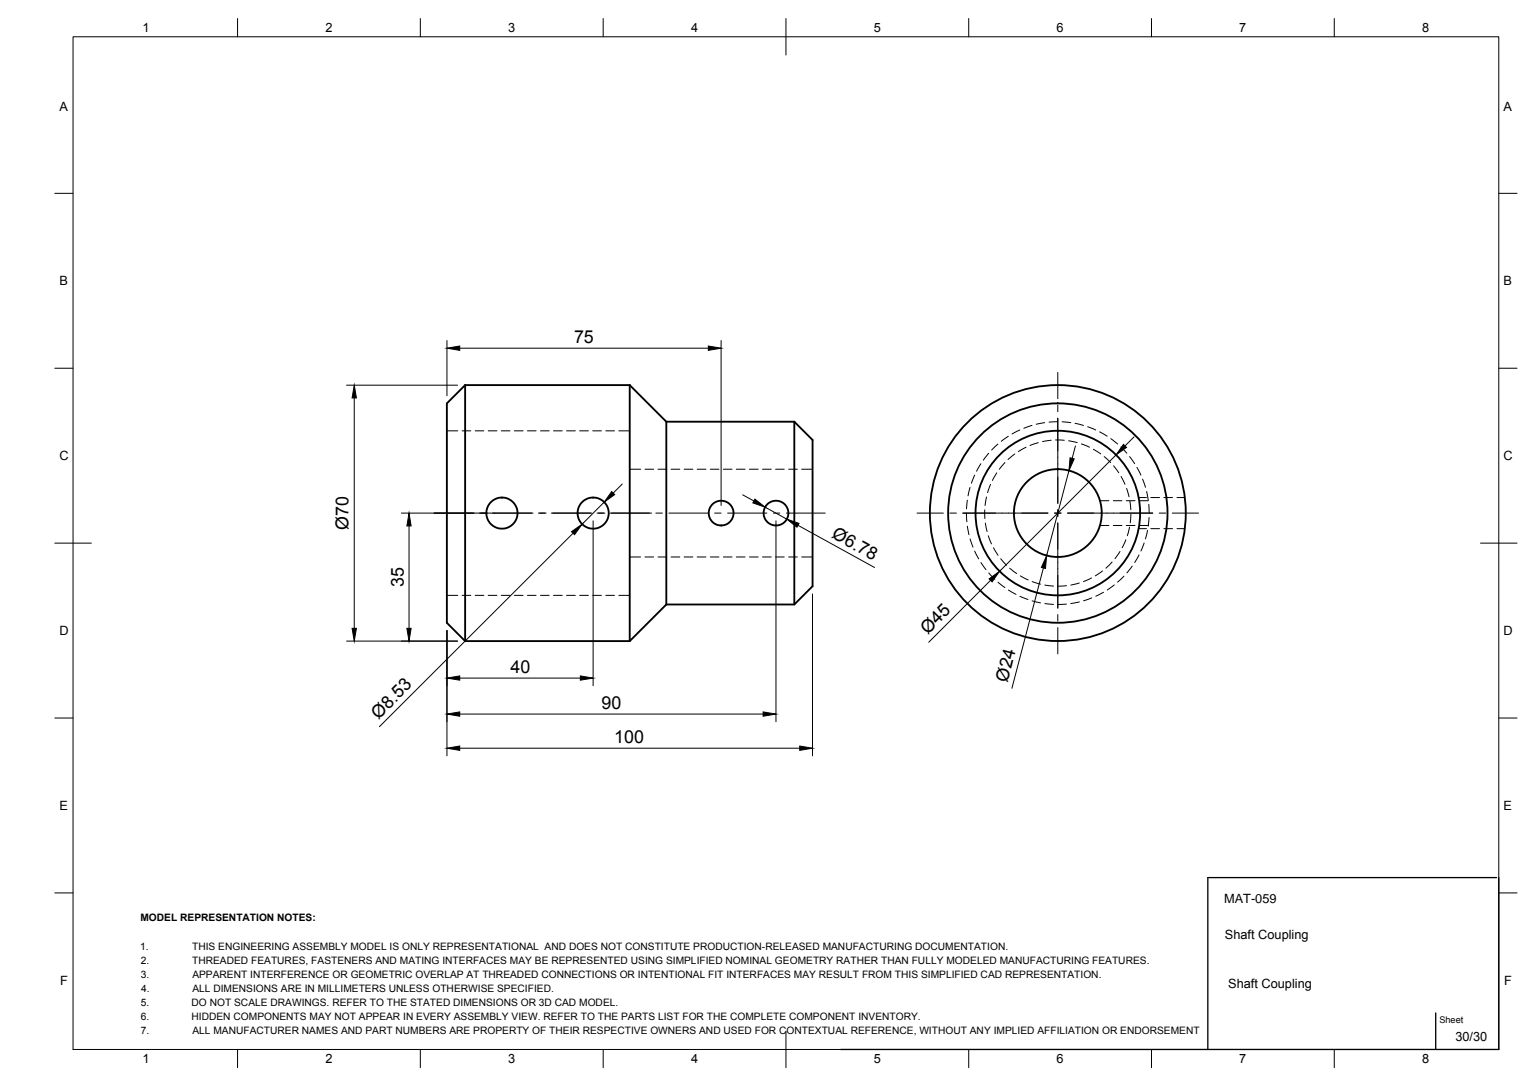
ISO-10303-21;
HEADER;
/* Generated by software containing ST-Developer
 * from STEP Tools, Inc. (www.steptools.com) 
 */

FILE_DESCRIPTION(
/* description */ ('', 'CAx-IF Rec.Pracs.---Representation and Presentation of Product Manufa
cturing Information (PMI)---4.0---2014-10-13'),
/* implementation_level */ '2;1');

FILE_NAME(
/* name */ 'Shaft Coupling.step',
/* time_stamp */ '2026-10-28T23:00:48+01:00',
/* author */ (''),
/* organization */ (''),
/* preprocessor_version */ 'ST-DEVELOPER v20.2',
/* originating_system */ 'Autodesk Translation Framework v15.17.0.0',
/* authorisation */ '');

FILE_SCHEMA (('AP242_MANAGED_MODEL_BASED_3D_ENGINEERING_MIM_LF { 1 0 10303 442 2 1 4 }'));
ENDSEC;

DATA;
#10=MECHANICAL_DESIGN_GEOMETRIC_PRESENTATION_REPRESENTATION('',(#999),#61811);
#707=CONICAL_SURFACE('',#38104,20.4999999999999,0.785398163397433);
#708=CONICAL_SURFACE('',#38107,30.4999999999998,0.785398163397455);
#709=CONICAL_SURFACE('',#38115,26.0000000000003,0.785398163397453);
#844=B_SPLINE_CURVE_WITH_KNOTS('',3,(#61360,#61361,#61362,#61363,#61364,
#61365,#61366,#61367,#61368,#61369,#61370,#61371,#61372,#61373,#61374,#61375,
#61376,#61377,#61378,#61379,#61380,#61381,#61382,#61383,#61384,#61385,#61386,
#61387,#61388,#61389,#61390,#61391,#61392,#61393),.UNSPECIFIED.,.T.,.F.,
(4,2,2,2,2,2,2,2,2,2,2,2,2,2,2,2,4),(-2.05511901424686,-1.92665918665082,
-1.79819935905478,-1.66976930986996,-1.54133926068514,-1.41290921150033,
-1.28447916231551,-1.15601933471947,-1.02755950712343,-0.899099679527391,
-0.770639851931354,-0.642209802746534,-0.513779753561715,-0.385349704376896,
-0.256919655192076,-0.128459827596038,0.),.UNSPECIFIED.);
#845=B_SPLINE_CURVE_WITH_KNOTS('',3,(#61395,#61396,#61397,#61398,#61399,
#61400,#61401,#61402,#61403,#61404,#61405,#61406,#61407,#61408,#61409,#61410,
#61411,#61412,#61413,#61414,#61415,#61416,#61417,#61418,#61419,#61420,#61421,
#61422,#61423,#61424,#61425,#61426,#61427,#61428),.UNSPECIFIED.,.T.,.F.,
(4,2,2,2,2,2,2,2,2,2,2,2,2,2,2,2,4),(-2.05511901424684,-1.9266591866508,
-1.79819935905477,-1.66976930986995,-1.54133926068513,-1.41290921150031,
-1.2844791623155,-1.15601933471946,-1.02755950712342,-0.899099679527382,
-0.770639851931344,-0.642209802746527,-0.513779753561709,-0.385349704376891,
-0.256919655192072,-0.128459827596036,0.),.UNSPECIFIED.);
#846=B_SPLINE_CURVE_WITH_KNOTS('',3,(#61431,#61432,#61433,#61434,#61435,
#61436,#61437,#61438,#61439,#61440,#61441,#61442,#61443,#61444,#61445,#61446,
#61447,#61448,#61449,#61450,#61451,#61452,#61453,#61454,#61455,#61456,#61457,
#61458,#61459,#61460,#61461,#61462,#61463,#61464),.UNSPECIFIED.,.T.,.F.,
(4,2,2,2,2,2,2,2,2,2,2,2,2,2,2,2,4),(-2.57601194234862,-2.41500757713331,
-2.254003211918,-2.09300608433973,-1.93200895676147,-1.7710118291832,-1.61001470160494,
-1.44901033638962,-1.28800597117431,-1.127001605959,-0.965997240743687,
-0.805000113165422,-0.644002985587156,-0.483005858008892,-0.322008730430627,
-0.161004365215313,0.),.UNSPECIFIED.);
#847=B_SPLINE_CURVE_WITH_KNOTS('',3,(#61467,#61468,#61469,#61470,#61471,
#61472,#61473,#61474,#61475,#61476,#61477,#61478,#61479,#61480,#61481,#61482,
#61483,#61484,#61485,#61486,#61487,#61488,#61489,#61490,#61491,#61492,#61493,
#61494,#61495,#61496,#61497,#61498,#61499,#61500),.UNSPECIFIED.,.T.,.F.,
(4,2,2,2,2,2,2,2,2,2,2,2,2,2,2,2,4),(0.,0.160753606357945,0.321507212715889,
0.4822596093528,0.643012005989711,0.803764402626621,0.964516799263531,1.12527040562148,
1.28602401197942,1.44677761833737,1.60753122469531,1.76828362133222,1.92903601796913,
2.08978841460604,2.25054081124296,2.4112944176009,2.57204802395885),
 .UNSPECIFIED.);
#848=B_SPLINE_CURVE_WITH_KNOTS('',3,(#61503,#61504,#61505,#61506,#61507,
#61508,#61509,#61510,#61511,#61512,#61513,#61514,#61515,#61516,#61517,#61518,
#61519,#61520,#61521,#61522,#61523,#61524,#61525,#61526,#61527,#61528,#61529,
#61530,#61531,#61532,#61533,#61534,#61535,#61536),.UNSPECIFIED.,.T.,.F.,
(4,2,2,2,2,2,2,2,2,2,2,2,2,2,2,2,4),(-2.57601194234859,-2.41500757713328,
-2.25400321191797,-2.09300608433971,-1.93200895676145,-1.77101182918318,
-1.61001470160492,-1.44901033638961,-1.2880059711743,-1.12700160595899,
-0.965997240743677,-0.805000113165413,-0.644002985587149,-0.483005858008886,
-0.322008730430623,-0.161004365215312,0.),.UNSPECIFIED.);
#849=B_SPLINE_CURVE_WITH_KNOTS('',3,(#61539,#61540,#61541,#61542,#61543,
#61544,#61545,#61546,#61547,#61548,#61549,#61550,#61551,#61552,#61553,#61554,
#61555,#61556,#61557,#61558,#61559,#61560,#61561,#61562,#61563,#61564,#61565,
#61566,#61567,#61568,#61569,#61570,#61571,#61572),.UNSPECIFIED.,.T.,.F.,
(4,2,2,2,2,2,2,2,2,2,2,2,2,2,2,2,4),(0.,0.160753606357943,0.321507212715886,
0.482259609352795,0.643012005989704,0.803764402626612,0.964516799263521,
1.12527040562146,1.28602401197941,1.44677761833735,1.60753122469529,1.7682836213322,
1.92903601796911,2.08978841460602,2.25054081124293,2.41129441760087,2.57204802395882),
 .UNSPECIFIED.);
#850=B_SPLINE_CURVE_WITH_KNOTS('',3,(#61577,#61578,#61579,#61580,#61581,
#61582,#61583,#61584,#61585,#61586,#61587,#61588,#61589,#61590,#61591,#61592,
#61593,#61594),.UNSPECIFIED.,.F.,.F.,(4,2,2,2,2,2,2,2,4),(0.,0.127857366097431,
0.255714732194861,0.383570615681227,0.511426499167593,0.639282382653959,
0.767138266140325,0.894995632237756,1.02285299833519),.UNSPECIFIED.);
#851=B_SPLINE_CURVE_WITH_KNOTS('',3,(#61595,#61596,#61597,#61598,#61599,
#61600,#61601,#61602,#61603,#61604,#61605,#61606,#61607,#61608,#61609,#61610,
#61611,#61612),.UNSPECIFIED.,.F.,.F.,(4,2,2,2,2,2,2,2,4),(1.02285299833519,
1.15071036443262,1.27856773053005,1.40642361401641,1.53427949750278,1.66213538098915,
1.78999126447551,1.91784863057294,2.04570599667037),.UNSPECIFIED.);
#852=B_SPLINE_CURVE_WITH_KNOTS('',3,(#61617,#61618,#61619,#61620,#61621,
#61622,#61623,#61624,#61625,#61626,#61627,#61628,#61629,#61630,#61631,#61632,
#61633,#61634),.UNSPECIFIED.,.F.,.F.,(4,2,2,2,2,2,2,2,4),(0.,0.12785736609743,
0.255714732194861,0.383570615681225,0.511426499167589,0.639282382653953,
0.767138266140317,0.894995632237748,1.02285299833518),.UNSPECIFIED.);
#853=B_SPLINE_CURVE_WITH_KNOTS('',3,(#61635,#61636,#61637,#61638,#61639,
#61640,#61641,#61642,#61643,#61644,#61645,#61646,#61647,#61648,#61649,#61650,
#61651,#61652),.UNSPECIFIED.,.F.,.F.,(4,2,2,2,2,2,2,2,4),(1.02285299833518,
1.15071036443261,1.27856773053004,1.4064236140164,1.53427949750277,1.66213538098913,
1.7899912644755,1.91784863057293,2.04570599667036),.UNSPECIFIED.);
#935=SHAPE_REPRESENTATION_RELATIONSHIP('SRR','None',#61997,#960);
#960=ADVANCED_BREP_SHAPE_REPRESENTATION('',(#1037),#61810);
#999=STYLED_ITEM('',(#62156),#1037);
#1037=MANIFOLD_SOLID_BREP('Body1',#33839);
#1870=CYLINDRICAL_SURFACE('',#38088,12.);
#1871=CYLINDRICAL_SURFACE('',#38091,4.26299999999998);
#1872=CYLINDRICAL_SURFACE('',#38092,4.26299999999993);
#1873=CYLINDRICAL_SURFACE('',#38093,3.38975000000002);
#1874=CYLINDRICAL_SURFACE('',#38094,3.38974999999999);
#1875=CYLINDRICAL_SURFACE('',#38097,22.5);
#1876=CYLINDRICAL_SURFACE('',#38099,24.9999999999999);
#1877=CYLINDRICAL_SURFACE('',#38111,35.0000000000001);
#2225=FACE_BOUND('',#8322,.T.);
#2226=FACE_BOUND('',#8323,.T.);
#2227=FACE_BOUND('',#8329,.T.);
#2228=FACE_BOUND('',#8331,.T.);
#2229=FACE_BOUND('',#8332,.T.);
#2230=FACE_BOUND('',#8334,.T.);
#2231=FACE_BOUND('',#8335,.T.);
#2232=FACE_BOUND('',#8338,.T.);
#2233=FACE_BOUND('',#8341,.T.);
#2234=FACE_BOUND('',#8342,.T.);
#2235=FACE_BOUND('',#8344,.T.);
#4218=CIRCLE('',#38089,12.);
#4219=CIRCLE('',#38090,12.);
#4220=CIRCLE('',#38096,22.5);
#4221=CIRCLE('',#38098,22.5);
#4222=CIRCLE('',#38100,25.);
#4223=CIRCLE('',#38101,25.);
#4224=CIRCLE('',#38102,25.);
#4225=CIRCLE('',#38103,25.);
#4226=CIRCLE('',#38105,20.);
#4227=CIRCLE('',#38108,35.);
#4228=CIRCLE('',#38109,35.);
#4229=CIRCLE('',#38110,29.9999999999998);
#4230=CIRCLE('',#38112,35.0000000000001);
#4231=CIRCLE('',#38113,35.0000000000001);
#6096=FACE_OUTER_BOUND('',#8321,.T.);
#6097=FACE_OUTER_BOUND('',#8324,.T.);
#6098=FACE_OUTER_BOUND('',#8325,.T.);
#6099=FACE_OUTER_BOUND('',#8326,.T.);
#6100=FACE_OUTER_BOUND('',#8327,.T.);
#6101=FACE_OUTER_BOUND('',#8328,.T.);
#6102=FACE_OUTER_BOUND('',#8330,.T.);
#6103=FACE_OUTER_BOUND('',#8333,.T.);
#6104=FACE_OUTER_BOUND('',#8336,.T.);
#6105=FACE_OUTER_BOUND('',#8337,.T.);
#6106=FACE_OUTER_BOUND('',#8339,.T.);
#6107=FACE_OUTER_BOUND('',#8340,.T.);
#6108=FACE_OUTER_BOUND('',#8343,.T.);
#6109=FACE_OUTER_BOUND('',#8345,.T.);
#8321=EDGE_LOOP('',(#31042,#31043,#31044,#31045));
#8322=EDGE_LOOP('',(#31046));
#8323=EDGE_LOOP('',(#31047));
#8324=EDGE_LOOP('',(#31048,#31049,#31050,#31051));
#8325=EDGE_LOOP('',(#31052,#31053,#31054,#31055));
#8326=EDGE_LOOP('',(#31056,#31057,#31058,#31059,#31060));
#8327=EDGE_LOOP('',(#31061,#31062,#31063,#31064,#31065));
#8328=EDGE_LOOP('',(#31066));
#8329=EDGE_LOOP('',(#31067));
#8330=EDGE_LOOP('',(#31068,#31069,#31070,#31071));
#8331=EDGE_LOOP('',(#31072));
#8332=EDGE_LOOP('',(#31073));
#8333=EDGE_LOOP('',(#31074,#31075,#31076,#31077,#31078,#31079));
#8334=EDGE_LOOP('',(#31080,#31081));
#8335=EDGE_LOOP('',(#31082,#31083));
#8336=EDGE_LOOP('',(#31084,#31085,#31086,#31087,#31088));
#8337=EDGE_LOOP('',(#31089));
#8338=EDGE_LOOP('',(#31090));
#8339=EDGE_LOOP('',(#31091,#31092,#31093,#31094,#31095));
#8340=EDGE_LOOP('',(#31096,#31097,#31098,#31099,#31100,#31101));
#8341=EDGE_LOOP('',(#31102));
#8342=EDGE_LOOP('',(#31103));
#8343=EDGE_LOOP('',(#31104));
#8344=EDGE_LOOP('',(#31105));
#8345=EDGE_LOOP('',(#31106,#31107,#31108,#31109,#31110,#31111));
#10882=LINE('',#61357,#13429);
#10883=LINE('',#61466,#13430);
#10884=LINE('',#61538,#13431);
#10885=LINE('',#61575,#13432);
#10886=LINE('',#61615,#13433);
#10887=LINE('',#61658,#13434);
#10888=LINE('',#61666,#13435);
#10889=LINE('',#61672,#13436);
#10890=LINE('',#61681,#13437);
#10891=LINE('',#61685,#13438);
#10892=LINE('',#61691,#13439);
#13429=VECTOR('',#48658,12.);
#13430=VECTOR('',#48663,4.26299999999998);
#13431=VECTOR('',#48666,4.26299999999993);
#13432=VECTOR('',#48669,3.38975000000002);
#13433=VECTOR('',#48672,3.38974999999999);
#13434=VECTOR('',#48679,22.5);
#13435=VECTOR('',#48688,24.9999999999999);
#13436=VECTOR('',#48695,20.4999999999999);
#13437=VECTOR('',#48706,30.4999999999998);
#13438=VECTOR('',#48711,35.0000000000001);
#13439=VECTOR('',#48720,26.0000000000003);
#16607=VERTEX_POINT('',#61354);
#16608=VERTEX_POINT('',#61356);
#16609=VERTEX_POINT('',#61359);
#16610=VERTEX_POINT('',#61394);
#16611=VERTEX_POINT('',#61430);
#16612=VERTEX_POINT('',#61465);
#16613=VERTEX_POINT('',#61502);
#16614=VERTEX_POINT('',#61537);
#16615=VERTEX_POINT('',#61574);
#16616=VERTEX_POINT('',#61576);
#16617=VERTEX_POINT('',#61614);
#16618=VERTEX_POINT('',#61616);
#16619=VERTEX_POINT('',#61654);
#16620=VERTEX_POINT('',#61657);
#16621=VERTEX_POINT('',#61661);
#16622=VERTEX_POINT('',#61662);
#16623=VERTEX_POINT('',#61665);
#16624=VERTEX_POINT('',#61667);
#16625=VERTEX_POINT('',#61671);
#16626=VERTEX_POINT('',#61676);
#16627=VERTEX_POINT('',#61677);
#16628=VERTEX_POINT('',#61680);
#16629=VERTEX_POINT('',#61684);
#16630=VERTEX_POINT('',#61686);
#21423=EDGE_CURVE('',#16607,#16607,#4218,.T.);
#21424=EDGE_CURVE('',#16607,#16608,#10882,.T.);
#21425=EDGE_CURVE('',#16608,#16608,#4219,.T.);
#21426=EDGE_CURVE('',#16609,#16609,#844,.T.);
#21427=EDGE_CURVE('',#16610,#16610,#845,.T.);
#21428=EDGE_CURVE('',#16611,#16611,#846,.T.);
#21429=EDGE_CURVE('',#16611,#16612,#10883,.T.);
#21430=EDGE_CURVE('',#16612,#16612,#847,.T.);
#21431=EDGE_CURVE('',#16613,#16613,#848,.T.);
#21432=EDGE_CURVE('',#16613,#16614,#10884,.T.);
#21433=EDGE_CURVE('',#16614,#16614,#849,.T.);
#21434=EDGE_CURVE('',#16609,#16615,#10885,.T.);
#21435=EDGE_CURVE('',#16616,#16615,#850,.T.);
#21436=EDGE_CURVE('',#16615,#16616,#851,.T.);
#21437=EDGE_CURVE('',#16610,#16617,#10886,.T.);
#21438=EDGE_CURVE('',#16618,#16617,#852,.T.);
#21439=EDGE_CURVE('',#16617,#16618,#853,.T.);
#21440=EDGE_CURVE('',#16619,#16619,#4220,.T.);
#21441=EDGE_CURVE('',#16619,#16620,#10887,.T.);
#21442=EDGE_CURVE('',#16620,#16620,#4221,.T.);
#21443=EDGE_CURVE('',#16621,#16622,#4222,.T.);
#21444=EDGE_CURVE('',#16622,#16621,#4223,.T.);
#21445=EDGE_CURVE('',#16622,#16623,#10888,.T.);
#21446=EDGE_CURVE('',#16624,#16623,#4224,.T.);
#21447=EDGE_CURVE('',#16623,#16624,#4225,.T.);
#21448=EDGE_CURVE('',#16621,#16625,#10889,.T.);
#21449=EDGE_CURVE('',#16625,#16625,#4226,.T.);
#21450=EDGE_CURVE('',#16626,#16627,#4227,.T.);
#21451=EDGE_CURVE('',#16627,#16626,#4228,.T.);
#21452=EDGE_CURVE('',#16626,#16628,#10890,.T.);
#21453=EDGE_CURVE('',#16628,#16628,#4229,.T.);
#21454=EDGE_CURVE('',#16627,#16629,#10891,.T.);
#21455=EDGE_CURVE('',#16630,#16629,#4230,.T.);
#21456=EDGE_CURVE('',#16629,#16630,#4231,.T.);
#21457=EDGE_CURVE('',#16630,#16624,#10892,.T.);
#31042=ORIENTED_EDGE('',*,*,#21423,.F.);
#31043=ORIENTED_EDGE('',*,*,#21424,.T.);
#31044=ORIENTED_EDGE('',*,*,#21425,.F.);
#31045=ORIENTED_EDGE('',*,*,#21424,.F.);
#31046=ORIENTED_EDGE('',*,*,#21426,.F.);
#31047=ORIENTED_EDGE('',*,*,#21427,.F.);
#31048=ORIENTED_EDGE('',*,*,#21428,.F.);
#31049=ORIENTED_EDGE('',*,*,#21429,.T.);
#31050=ORIENTED_EDGE('',*,*,#21430,.F.);
#31051=ORIENTED_EDGE('',*,*,#21429,.F.);
#31052=ORIENTED_EDGE('',*,*,#21431,.F.);
#31053=ORIENTED_EDGE('',*,*,#21432,.T.);
#31054=ORIENTED_EDGE('',*,*,#21433,.F.);
#31055=ORIENTED_EDGE('',*,*,#21432,.F.);
#31056=ORIENTED_EDGE('',*,*,#21426,.T.);
#31057=ORIENTED_EDGE('',*,*,#21434,.T.);
#31058=ORIENTED_EDGE('',*,*,#21435,.F.);
#31059=ORIENTED_EDGE('',*,*,#21436,.F.);
#31060=ORIENTED_EDGE('',*,*,#21434,.F.);
#31061=ORIENTED_EDGE('',*,*,#21427,.T.);
#31062=ORIENTED_EDGE('',*,*,#21437,.T.);
#31063=ORIENTED_EDGE('',*,*,#21438,.F.);
#31064=ORIENTED_EDGE('',*,*,#21439,.F.);
#31065=ORIENTED_EDGE('',*,*,#21437,.F.);
#31066=ORIENTED_EDGE('',*,*,#21440,.T.);
#31067=ORIENTED_EDGE('',*,*,#21425,.T.);
#31068=ORIENTED_EDGE('',*,*,#21440,.F.);
#31069=ORIENTED_EDGE('',*,*,#21441,.T.);
#31070=ORIENTED_EDGE('',*,*,#21442,.F.);
#31071=ORIENTED_EDGE('',*,*,#21441,.F.);
#31072=ORIENTED_EDGE('',*,*,#21428,.T.);
#31073=ORIENTED_EDGE('',*,*,#21431,.T.);
#31074=ORIENTED_EDGE('',*,*,#21443,.F.);
#31075=ORIENTED_EDGE('',*,*,#21444,.F.);
#31076=ORIENTED_EDGE('',*,*,#21445,.T.);
#31077=ORIENTED_EDGE('',*,*,#21446,.F.);
#31078=ORIENTED_EDGE('',*,*,#21447,.F.);
#31079=ORIENTED_EDGE('',*,*,#21445,.F.);
#31080=ORIENTED_EDGE('',*,*,#21435,.T.);
#31081=ORIENTED_EDGE('',*,*,#21436,.T.);
#31082=ORIENTED_EDGE('',*,*,#21438,.T.);
#31083=ORIENTED_EDGE('',*,*,#21439,.T.);
#31084=ORIENTED_EDGE('',*,*,#21443,.T.);
#31085=ORIENTED_EDGE('',*,*,#21444,.T.);
#31086=ORIENTED_EDGE('',*,*,#21448,.T.);
#31087=ORIENTED_EDGE('',*,*,#21449,.T.);
#31088=ORIENTED_EDGE('',*,*,#21448,.F.);
#31089=ORIENTED_EDGE('',*,*,#21449,.F.);
#31090=ORIENTED_EDGE('',*,*,#21423,.T.);
#31091=ORIENTED_EDGE('',*,*,#21450,.T.);
#31092=ORIENTED_EDGE('',*,*,#21451,.T.);
#31093=ORIENTED_EDGE('',*,*,#21452,.T.);
#31094=ORIENTED_EDGE('',*,*,#21453,.T.);
#31095=ORIENTED_EDGE('',*,*,#21452,.F.);
#31096=ORIENTED_EDGE('',*,*,#21450,.F.);
#31097=ORIENTED_EDGE('',*,*,#21451,.F.);
#31098=ORIENTED_EDGE('',*,*,#21454,.T.);
#31099=ORIENTED_EDGE('',*,*,#21455,.F.);
#31100=ORIENTED_EDGE('',*,*,#21456,.F.);
#31101=ORIENTED_EDGE('',*,*,#21454,.F.);
#31102=ORIENTED_EDGE('',*,*,#21430,.T.);
#31103=ORIENTED_EDGE('',*,*,#21433,.T.);
#31104=ORIENTED_EDGE('',*,*,#21453,.F.);
#31105=ORIENTED_EDGE('',*,*,#21442,.T.);
#31106=ORIENTED_EDGE('',*,*,#21456,.T.);
#31107=ORIENTED_EDGE('',*,*,#21457,.T.);
#31108=ORIENTED_EDGE('',*,*,#21446,.T.);
#31109=ORIENTED_EDGE('',*,*,#21447,.T.);
#31110=ORIENTED_EDGE('',*,*,#21457,.F.);
#31111=ORIENTED_EDGE('',*,*,#21455,.T.);
#31910=PLANE('',#38095);
#31911=PLANE('',#38106);
#31912=PLANE('',#38114);
#33777=ADVANCED_FACE('',(#6096,#2225,#2226),#1870,.F.);
#33778=ADVANCED_FACE('',(#6097),#1871,.F.);
#33779=ADVANCED_FACE('',(#6098),#1872,.F.);
#33780=ADVANCED_FACE('',(#6099),#1873,.F.);
#33781=ADVANCED_FACE('',(#6100),#1874,.F.);
#33782=ADVANCED_FACE('',(#6101,#2227),#31910,.T.);
#33783=ADVANCED_FACE('',(#6102,#2228,#2229),#1875,.F.);
#33784=ADVANCED_FACE('',(#6103,#2230,#2231),#1876,.T.);
#33785=ADVANCED_FACE('',(#6104),#707,.T.);
#33786=ADVANCED_FACE('',(#6105,#2232),#31911,.T.);
#33787=ADVANCED_FACE('',(#6106),#708,.T.);
#33788=ADVANCED_FACE('',(#6107,#2233,#2234),#1877,.T.);
#33789=ADVANCED_FACE('',(#6108,#2235),#31912,.T.);
#33790=ADVANCED_FACE('',(#6109),#709,.T.);
#33839=CLOSED_SHELL('',(#33777,#33778,#33779,#33780,#33781,#33782,#33783,
#33784,#33785,#33786,#33787,#33788,#33789,#33790));
#38087=AXIS2_PLACEMENT_3D('',#61352,#48652,#48653);
#38088=AXIS2_PLACEMENT_3D('',#61353,#48654,#48655);
#38089=AXIS2_PLACEMENT_3D('',#61355,#48656,#48657);
#38090=AXIS2_PLACEMENT_3D('',#61358,#48659,#48660);
#38091=AXIS2_PLACEMENT_3D('',#61429,#48661,#48662);
#38092=AXIS2_PLACEMENT_3D('',#61501,#48664,#48665);
#38093=AXIS2_PLACEMENT_3D('',#61573,#48667,#48668);
#38094=AXIS2_PLACEMENT_3D('',#61613,#48670,#48671);
#38095=AXIS2_PLACEMENT_3D('',#61653,#48673,#48674);
#38096=AXIS2_PLACEMENT_3D('',#61655,#48675,#48676);
#38097=AXIS2_PLACEMENT_3D('',#61656,#48677,#48678);
#38098=AXIS2_PLACEMENT_3D('',#61659,#48680,#48681);
#38099=AXIS2_PLACEMENT_3D('',#61660,#48682,#48683);
#38100=AXIS2_PLACEMENT_3D('',#61663,#48684,#48685);
#38101=AXIS2_PLACEMENT_3D('',#61664,#48686,#48687);
#38102=AXIS2_PLACEMENT_3D('',#61668,#48689,#48690);
#38103=AXIS2_PLACEMENT_3D('',#61669,#48691,#48692);
#38104=AXIS2_PLACEMENT_3D('',#61670,#48693,#48694);
#38105=AXIS2_PLACEMENT_3D('',#61673,#48696,#48697);
#38106=AXIS2_PLACEMENT_3D('',#61674,#48698,#48699);
#38107=AXIS2_PLACEMENT_3D('',#61675,#48700,#48701);
#38108=AXIS2_PLACEMENT_3D('',#61678,#48702,#48703);
#38109=AXIS2_PLACEMENT_3D('',#61679,#48704,#48705);
#38110=AXIS2_PLACEMENT_3D('',#61682,#48707,#48708);
#38111=AXIS2_PLACEMENT_3D('',#61683,#48709,#48710);
#38112=AXIS2_PLACEMENT_3D('',#61687,#48712,#48713);
#38113=AXIS2_PLACEMENT_3D('',#61688,#48714,#48715);
#38114=AXIS2_PLACEMENT_3D('',#61689,#48716,#48717);
#38115=AXIS2_PLACEMENT_3D('',#61690,#48718,#48719);
#48652=DIRECTION('axis',(0.,0.,1.));
#48653=DIRECTION('refdir',(1.,0.,0.));
#48654=DIRECTION('center_axis',(-7.56024872335536E-14,1.,-6.79969489730031E-15));
#48655=DIRECTION('ref_axis',(-1.,-7.56024872335536E-14,-2.77555756156749E-16));
#48656=DIRECTION('center_axis',(-7.56239704097264E-14,1.,-6.79973512277291E-15));
#48657=DIRECTION('ref_axis',(-1.,-7.56239704097264E-14,-2.77555756156749E-16));
#48658=DIRECTION('',(-7.56024872335536E-14,1.,-6.79969489730031E-15));
#48659=DIRECTION('center_axis',(6.72435353857335E-14,-1.,5.37013150103301E-15));
#48660=DIRECTION('ref_axis',(-1.,-6.72435353857335E-14,-2.77555756156794E-16));
#48661=DIRECTION('center_axis',(-2.7755575615629E-16,-6.07241588737381E-15,
1.));
#48662=DIRECTION('ref_axis',(-1.,-1.66533453693771E-16,-2.77555756156291E-16));
#48663=DIRECTION('',(-2.7755575615629E-16,-6.07241588737381E-15,1.));
#48664=DIRECTION('center_axis',(-2.7755575615629E-16,-6.07241588737381E-15,
1.));
#48665=DIRECTION('ref_axis',(-1.,-1.66533453693771E-16,-2.77555756156291E-16));
#48666=DIRECTION('',(-2.7755575615629E-16,-6.07241588737381E-15,1.));
#48667=DIRECTION('center_axis',(-2.7755575615629E-16,-6.07241588737381E-15,
1.));
#48668=DIRECTION('ref_axis',(-1.,-1.66533453693771E-16,-2.77555756156291E-16));
#48669=DIRECTION('',(-2.7755575615629E-16,-6.07241588737381E-15,1.));
#48670=DIRECTION('center_axis',(-2.7755575615629E-16,-6.07241588737381E-15,
1.));
#48671=DIRECTION('ref_axis',(-1.,-1.66533453693771E-16,-2.77555756156291E-16));
#48672=DIRECTION('',(-2.7755575615629E-16,-6.07241588737381E-15,1.));
#48673=DIRECTION('center_axis',(-6.72435353857335E-14,1.,-5.37013150103301E-15));
#48674=DIRECTION('ref_axis',(-2.77555756156297E-16,5.37013150103299E-15,
1.));
#48675=DIRECTION('center_axis',(-7.25862069473908E-14,1.,-6.26042944676291E-15));
#48676=DIRECTION('ref_axis',(-0.813826036051072,-6.27105343449563E-14,-0.581108581114923));
#48677=DIRECTION('center_axis',(-7.40629779727442E-14,1.,-6.07998716438531E-15));
#48678=DIRECTION('ref_axis',(-1.,-7.40629779727442E-14,-2.77555756156744E-16));
#48679=DIRECTION('',(-7.40629779727442E-14,1.,-6.07998716438531E-15));
#48680=DIRECTION('center_axis',(6.87609227137152E-14,-1.,-8.76572429925892E-16));
#48681=DIRECTION('ref_axis',(-0.813826036051074,-5.64688129283158E-14,0.581108581114921));
#48682=DIRECTION('center_axis',(7.42659901829614E-14,-1.,6.84057719202601E-15));
#48683=DIRECTION('ref_axis',(-1.,-7.42659901829614E-14,-2.77555756156738E-16));
#48684=DIRECTION('center_axis',(7.5080331238299E-14,-1.,-7.2741312686569E-16));
#48685=DIRECTION('ref_axis',(-0.813826036051074,-6.15250343671038E-14,0.58110858111492));
#48686=DIRECTION('center_axis',(7.5080331238299E-14,-1.,-7.2741312686569E-16));
#48687=DIRECTION('ref_axis',(-0.813826036051074,-6.15250343671038E-14,0.58110858111492));
#48688=DIRECTION('',(-7.42659901829614E-14,1.,-6.84057719202601E-15));
#48689=DIRECTION('center_axis',(-8.11684053303452E-14,1.,-3.37179773151922E-14));
#48690=DIRECTION('ref_axis',(-1.,-8.11684053303452E-14,-9.06219543850778E-16));
#48691=DIRECTION('center_axis',(-8.11684053303452E-14,1.,-3.37179773151922E-14));
#48692=DIRECTION('ref_axis',(-1.,-8.11684053303452E-14,-9.06219543850778E-16));
#48693=DIRECTION('center_axis',(-4.77076649660703E-14,1.,-1.51365987155128E-14));
#48694=DIRECTION('ref_axis',(-0.813826036051047,-4.76217472710665E-14,-0.581108581114958));
#48695=DIRECTION('',(-0.57546190879782,-0.707106781186592,-0.410905818312063));
#48696=DIRECTION('center_axis',(-7.86398561629848E-14,1.,1.45566060036366E-14));
#48697=DIRECTION('ref_axis',(-0.813826036051073,-5.55401937561262E-14,-0.581108581114922));
#48698=DIRECTION('center_axis',(7.56239704097264E-14,-1.,6.79973512277291E-15));
#48699=DIRECTION('ref_axis',(2.77555756156191E-16,-6.79973512277289E-15,
-1.));
#48700=DIRECTION('center_axis',(7.6307102664867E-14,-1.,1.38622525122371E-14));
#48701=DIRECTION('ref_axis',(-0.813826036051067,-5.40452329958475E-14,0.58110858111493));
#48702=DIRECTION('center_axis',(-7.39721188273472E-14,1.,-1.0554808768484E-16));
#48703=DIRECTION('ref_axis',(-0.813826036051073,-6.02617711430328E-14,-0.581108581114922));
#48704=DIRECTION('center_axis',(-7.39721188273472E-14,1.,-1.0554808768484E-16));
#48705=DIRECTION('ref_axis',(-0.813826036051073,-6.02617711430328E-14,-0.581108581114922));
#48706=DIRECTION('',(-0.575461908797935,0.707106781186504,0.410905818312053));
#48707=DIRECTION('center_axis',(6.7216128184098E-14,-1.,-3.09884788437082E-15));
#48708=DIRECTION('ref_axis',(-0.813826036051075,-5.65030022559431E-14,0.581108581114919));
#48709=DIRECTION('center_axis',(-6.6878601422281E-14,1.,-8.42209836172541E-15));
#48710=DIRECTION('ref_axis',(-1.,-6.6878601422281E-14,-9.81357852128142E-17));
#48711=DIRECTION('',(6.6878601422281E-14,-1.,8.42209836172541E-15));
#48712=DIRECTION('center_axis',(7.17283375552464E-14,-1.,6.61584725119951E-15));
#48713=DIRECTION('ref_axis',(-1.,-7.17283375552463E-14,5.75531685801174E-15));
#48714=DIRECTION('center_axis',(7.17283375552464E-14,-1.,6.61584725119951E-15));
#48715=DIRECTION('ref_axis',(-1.,-7.17283375552463E-14,5.75531685801174E-15));
#48716=DIRECTION('center_axis',(-8.30355629492075E-14,1.,-2.21448706217753E-15));
#48717=DIRECTION('ref_axis',(-2.77555756156507E-16,2.21448706217751E-15,
1.));
#48718=DIRECTION('center_axis',(-5.82747545344175E-14,1.,-7.72560328633601E-15));
#48719=DIRECTION('ref_axis',(0.813826036051082,5.19149268485742E-14,0.581108581114909));
#48720=DIRECTION('',(0.575461908797932,-0.707106781186507,0.410905818312053));
#61352=CARTESIAN_POINT('',(0.,0.,0.));
#61353=CARTESIAN_POINT('Origin',(375.115917770965,45.027992731211,445.000000551893));
#61354=CARTESIAN_POINT('',(387.115917770965,45.027992731212,445.000000551893));
#61355=CARTESIAN_POINT('Origin',(375.115917770965,45.027992731211,445.000000551893));
#61356=CARTESIAN_POINT('',(387.115917770961,95.027992731212,445.000000551892));
#61357=CARTESIAN_POINT('',(387.115917770965,45.0279927312119,445.000000551893));
#61358=CARTESIAN_POINT('Origin',(375.115917770961,95.027992731211,445.000000551892));
#61359=CARTESIAN_POINT('',(378.505667770963,70.0279927312109,456.511281755021));
#61360=CARTESIAN_POINT('Ctrl Pts',(378.505667770963,70.0279927312112,456.511281755021));
#61361=CARTESIAN_POINT('Ctrl Pts',(378.505667770963,69.599793305891,456.511281755021));
#61362=CARTESIAN_POINT('Ctrl Pts',(378.419612733572,69.1447595869222,456.537670683632));
#61363=CARTESIAN_POINT('Ctrl Pts',(378.07298028749,68.3103537068892,456.631338076663));
#61364=CARTESIAN_POINT('Ctrl Pts',(377.812518336597,67.9307628737902,456.697089455795));
#61365=CARTESIAN_POINT('Ctrl Pts',(377.213217098769,67.331461635963,456.819257533707));
#61366=CARTESIAN_POINT('Ctrl Pts',(376.833597772799,67.0709457470152,456.883844434558));
#61367=CARTESIAN_POINT('Ctrl Pts',(375.999089280567,66.7242736548161,456.974814875745));
#61368=CARTESIAN_POINT('Ctrl Pts',(375.544017934913,66.6382427312109,457.000000551892));
#61369=CARTESIAN_POINT('Ctrl Pts',(374.687817607014,66.6382427312109,457.000000551892));
#61370=CARTESIAN_POINT('Ctrl Pts',(374.23274626136,66.724273654816,456.974814875745));
#61371=CARTESIAN_POINT('Ctrl Pts',(373.398237769128,67.0709457470149,456.883844434558));
#61372=CARTESIAN_POINT('Ctrl Pts',(373.018618443157,67.3314616359627,456.819257533707));
#61373=CARTESIAN_POINT('Ctrl Pts',(372.41931720533,67.9307628737898,456.697089455795));
#61374=CARTESIAN_POINT('Ctrl Pts',(372.158855254436,68.3103537068888,456.631338076663));
#61375=CARTESIAN_POINT('Ctrl Pts',(371.812222808355,69.1447595869217,456.537670683632));
#61376=CARTESIAN_POINT('Ctrl Pts',(371.726167770963,69.5997933058905,456.511281755021));
#61377=CARTESIAN_POINT('Ctrl Pts',(371.726167770963,70.4561921565308,456.511281755021));
#61378=CARTESIAN_POINT('Ctrl Pts',(371.812222808355,70.9112258754996,456.537670683632));
#61379=CARTESIAN_POINT('Ctrl Pts',(372.158855254436,71.7456317555326,456.631338076663));
#61380=CARTESIAN_POINT('Ctrl Pts',(372.41931720533,72.1252225886316,456.697089455795));
#61381=CARTESIAN_POINT('Ctrl Pts',(373.018618443157,72.7245238264588,456.819257533707));
#61382=CARTESIAN_POINT('Ctrl Pts',(373.398237769127,72.9850397154067,456.883844434558));
#61383=CARTESIAN_POINT('Ctrl Pts',(374.232746261359,73.3317118076057,456.974814875745));
#61384=CARTESIAN_POINT('Ctrl Pts',(374.687817607013,73.4177427312109,457.000000551892));
#61385=CARTESIAN_POINT('Ctrl Pts',(375.544017934912,73.417742731211,457.000000551892));
#61386=CARTESIAN_POINT('Ctrl Pts',(375.999089280567,73.3317118076058,456.974814875745));
#61387=CARTESIAN_POINT('Ctrl Pts',(376.833597772799,72.9850397154069,456.883844434557));
#61388=CARTESIAN_POINT('Ctrl Pts',(377.213217098769,72.7245238264592,456.819257533707));
#61389=CARTESIAN_POINT('Ctrl Pts',(377.812518336596,72.125222588632,456.697089455795));
#61390=CARTESIAN_POINT('Ctrl Pts',(378.07298028749,71.7456317555331,456.631338076663));
#61391=CARTESIAN_POINT('Ctrl Pts',(378.419612733571,70.9112258755002,456.537670683632));
#61392=CARTESIAN_POINT('Ctrl Pts',(378.505667770963,70.4561921565313,456.511281755021));
#61393=CARTESIAN_POINT('Ctrl Pts',(378.505667770963,70.0279927312112,456.511281755021));
#61394=CARTESIAN_POINT('',(378.505667770964,55.027992731211,456.511281755021));
#61395=CARTESIAN_POINT('Ctrl Pts',(378.505667770964,55.0279927312112,456.511281755021));
#61396=CARTESIAN_POINT('Ctrl Pts',(378.505667770964,54.5997933058911,456.511281755021));
#61397=CARTESIAN_POINT('Ctrl Pts',(378.419612733573,54.1447595869223,456.537670683633));
#61398=CARTESIAN_POINT('Ctrl Pts',(378.072980287491,53.3103537068893,456.631338076663));
#61399=CARTESIAN_POINT('Ctrl Pts',(377.812518336598,52.9307628737903,456.697089455795));
#61400=CARTESIAN_POINT('Ctrl Pts',(377.213217098771,52.331461635963,456.819257533707));
#61401=CARTESIAN_POINT('Ctrl Pts',(376.8335977728,52.0709457470152,456.883844434558));
#61402=CARTESIAN_POINT('Ctrl Pts',(375.999089280568,51.7242736548162,456.974814875745));
#61403=CARTESIAN_POINT('Ctrl Pts',(375.544017934914,51.638242731211,457.000000551893));
#61404=CARTESIAN_POINT('Ctrl Pts',(374.687817607015,51.6382427312109,457.000000551893));
#61405=CARTESIAN_POINT('Ctrl Pts',(374.232746261361,51.7242736548161,456.974814875745));
#61406=CARTESIAN_POINT('Ctrl Pts',(373.398237769129,52.070945747015,456.883844434558));
#61407=CARTESIAN_POINT('Ctrl Pts',(373.018618443158,52.3314616359627,456.819257533707));
#61408=CARTESIAN_POINT('Ctrl Pts',(372.419317205331,52.9307628737898,456.697089455795));
#61409=CARTESIAN_POINT('Ctrl Pts',(372.158855254437,53.3103537068888,456.631338076663));
#61410=CARTESIAN_POINT('Ctrl Pts',(371.812222808356,54.1447595869217,456.537670683633));
#61411=CARTESIAN_POINT('Ctrl Pts',(371.726167770964,54.5997933058906,456.511281755021));
#61412=CARTESIAN_POINT('Ctrl Pts',(371.726167770964,55.4561921565308,456.511281755021));
#61413=CARTESIAN_POINT('Ctrl Pts',(371.812222808356,55.9112258754996,456.537670683633));
#61414=CARTESIAN_POINT('Ctrl Pts',(372.158855254437,56.7456317555326,456.631338076663));
#61415=CARTESIAN_POINT('Ctrl Pts',(372.419317205331,57.1252225886316,456.697089455795));
#61416=CARTESIAN_POINT('Ctrl Pts',(373.018618443158,57.7245238264589,456.819257533707));
#61417=CARTESIAN_POINT('Ctrl Pts',(373.398237769128,57.9850397154067,456.883844434558));
#61418=CARTESIAN_POINT('Ctrl Pts',(374.23274626136,58.3317118076057,456.974814875745));
#61419=CARTESIAN_POINT('Ctrl Pts',(374.687817607015,58.4177427312109,457.000000551893));
#61420=CARTESIAN_POINT('Ctrl Pts',(375.544017934913,58.417742731211,457.000000551893));
#61421=CARTESIAN_POINT('Ctrl Pts',(375.999089280568,58.3317118076058,456.974814875745));
#61422=CARTESIAN_POINT('Ctrl Pts',(376.8335977728,57.9850397154069,456.883844434558));
#61423=CARTESIAN_POINT('Ctrl Pts',(377.21321709877,57.7245238264592,456.819257533707));
#61424=CARTESIAN_POINT('Ctrl Pts',(377.812518336597,57.125222588632,456.697089455795));
#61425=CARTESIAN_POINT('Ctrl Pts',(378.072980287491,56.7456317555331,456.631338076663));
#61426=CARTESIAN_POINT('Ctrl Pts',(378.419612733572,55.9112258755001,456.537670683633));
#61427=CARTESIAN_POINT('Ctrl Pts',(378.505667770964,55.4561921565313,456.511281755021));
#61428=CARTESIAN_POINT('Ctrl Pts',(378.505667770964,55.0279927312112,456.511281755021));
#61429=CARTESIAN_POINT('Origin',(375.115917770959,129.966587529218,473.546231028847));
#61430=CARTESIAN_POINT('',(379.378917770959,129.966587529218,467.092461505801));
#61431=CARTESIAN_POINT('Ctrl Pts',(379.378917770959,129.966587529218,467.092461505801));
#61432=CARTESIAN_POINT('Ctrl Pts',(379.378917770959,130.503268746603,467.092461505801));
#61433=CARTESIAN_POINT('Ctrl Pts',(379.271395654013,131.074810160741,467.114043744988));
#61434=CARTESIAN_POINT('Ctrl Pts',(378.83594383252,132.124725811365,467.191447285196));
#61435=CARTESIAN_POINT('Ctrl Pts',(378.508082726548,132.603214990025,467.246090869443));
#61436=CARTESIAN_POINT('Ctrl Pts',(377.752562213622,133.358735502951,467.348231142275));
#61437=CARTESIAN_POINT('Ctrl Pts',(377.274065797272,133.686609917986,467.402443514309));
#61438=CARTESIAN_POINT('Ctrl Pts',(376.224125087311,134.122071395634,467.478855729964));
#61439=CARTESIAN_POINT('Ctrl Pts',(375.652574862886,134.229587529218,467.500000551892));
#61440=CARTESIAN_POINT('Ctrl Pts',(374.579260679031,134.229587529218,467.500000551892));
#61441=CARTESIAN_POINT('Ctrl Pts',(374.007710454606,134.122071395634,467.478855729964));
#61442=CARTESIAN_POINT('Ctrl Pts',(372.957769744645,133.686609917986,467.402443514309));
#61443=CARTESIAN_POINT('Ctrl Pts',(372.479273328295,133.35873550295,467.348231142275));
#61444=CARTESIAN_POINT('Ctrl Pts',(371.723752815369,132.603214990025,467.246090869443));
#61445=CARTESIAN_POINT('Ctrl Pts',(371.395891709397,132.124725811364,467.191447285196));
#61446=CARTESIAN_POINT('Ctrl Pts',(370.960439887904,131.074810160741,467.114043744988));
#61447=CARTESIAN_POINT('Ctrl Pts',(370.852917770959,130.503268746602,467.092461505801));
#61448=CARTESIAN_POINT('Ctrl Pts',(370.852917770959,129.429906311833,467.092461505801));
#61449=CARTESIAN_POINT('Ctrl Pts',(370.960439887905,128.858364897694,467.114043744988));
#61450=CARTESIAN_POINT('Ctrl Pts',(371.395891709398,127.808449247071,467.191447285196));
#61451=CARTESIAN_POINT('Ctrl Pts',(371.723752815369,127.329960068411,467.246090869443));
#61452=CARTESIAN_POINT('Ctrl Pts',(372.479273328295,126.574439555485,467.348231142275));
#61453=CARTESIAN_POINT('Ctrl Pts',(372.957769744646,126.24656514045,467.402443514309));
#61454=CARTESIAN_POINT('Ctrl Pts',(374.007710454607,125.811103662802,467.478855729964));
#61455=CARTESIAN_POINT('Ctrl Pts',(374.579260679031,125.703587529218,467.500000551892));
#61456=CARTESIAN_POINT('Ctrl Pts',(375.652574862887,125.703587529218,467.500000551892));
#61457=CARTESIAN_POINT('Ctrl Pts',(376.224125087311,125.811103662802,467.478855729964));
#61458=CARTESIAN_POINT('Ctrl Pts',(377.274065797272,126.24656514045,467.402443514309));
#61459=CARTESIAN_POINT('Ctrl Pts',(377.752562213623,126.574439555485,467.348231142275));
#61460=CARTESIAN_POINT('Ctrl Pts',(378.508082726548,127.329960068411,467.246090869443));
#61461=CARTESIAN_POINT('Ctrl Pts',(378.83594383252,127.808449247071,467.191447285196));
#61462=CARTESIAN_POINT('Ctrl Pts',(379.271395654013,128.858364897695,467.114043744988));
#61463=CARTESIAN_POINT('Ctrl Pts',(379.378917770959,129.429906311834,467.092461505801));
#61464=CARTESIAN_POINT('Ctrl Pts',(379.378917770959,129.966587529218,467.092461505801));
#61465=CARTESIAN_POINT('',(379.378917770959,129.966587529218,479.739413773764));
#61466=CARTESIAN_POINT('',(379.378917770959,129.966587529218,473.546231028847));
#61467=CARTESIAN_POINT('Ctrl Pts',(379.378917770959,129.966587529218,479.739413773764));
#61468=CARTESIAN_POINT('Ctrl Pts',(379.378917770959,129.430742174692,479.739413773764));
#61469=CARTESIAN_POINT('Ctrl Pts',(379.27171989715,128.859547272367,479.753090630837));
#61470=CARTESIAN_POINT('Ctrl Pts',(378.836500546947,127.809391754052,479.802374391123));
#61471=CARTESIAN_POINT('Ctrl Pts',(378.508507955967,127.33038529783,479.837256921998));
#61472=CARTESIAN_POINT('Ctrl Pts',(377.752122848375,126.574000190238,479.90264400738));
#61473=CARTESIAN_POINT('Ctrl Pts',(377.273115153634,126.246005370261,479.937413294597));
#61474=CARTESIAN_POINT('Ctrl Pts',(376.22295544681,125.810784382548,479.986437599388));
#61475=CARTESIAN_POINT('Ctrl Pts',(375.651759093082,125.703587529218,480.000000551892));
#61476=CARTESIAN_POINT('Ctrl Pts',(374.580076448836,125.703587529218,480.000000551892));
#61477=CARTESIAN_POINT('Ctrl Pts',(374.008880095108,125.810784382548,479.986437599388));
#61478=CARTESIAN_POINT('Ctrl Pts',(372.958720388284,126.246005370261,479.937413294597));
#61479=CARTESIAN_POINT('Ctrl Pts',(372.479712693543,126.574000190237,479.90264400738));
#61480=CARTESIAN_POINT('Ctrl Pts',(371.723327585951,127.330385297829,479.837256921998));
#61481=CARTESIAN_POINT('Ctrl Pts',(371.395334994971,127.809391754051,479.802374391123));
#61482=CARTESIAN_POINT('Ctrl Pts',(370.960115644768,128.859547272367,479.753090630837));
#61483=CARTESIAN_POINT('Ctrl Pts',(370.852917770959,129.430742174691,479.739413773764));
#61484=CARTESIAN_POINT('Ctrl Pts',(370.852917770959,130.502432883744,479.739413773764));
#61485=CARTESIAN_POINT('Ctrl Pts',(370.960115644767,131.073627786068,479.753090630837));
#61486=CARTESIAN_POINT('Ctrl Pts',(371.39533499497,132.123783304384,479.802374391123));
#61487=CARTESIAN_POINT('Ctrl Pts',(371.723327585951,132.602789760606,479.837256921998));
#61488=CARTESIAN_POINT('Ctrl Pts',(372.479712693542,133.359174868198,479.90264400738));
#61489=CARTESIAN_POINT('Ctrl Pts',(372.958720388284,133.687169688174,479.937413294597));
#61490=CARTESIAN_POINT('Ctrl Pts',(374.008880095108,134.122390675888,479.986437599388));
#61491=CARTESIAN_POINT('Ctrl Pts',(374.580076448835,134.229587529218,480.000000551892));
#61492=CARTESIAN_POINT('Ctrl Pts',(375.651759093081,134.229587529218,480.000000551892));
#61493=CARTESIAN_POINT('Ctrl Pts',(376.222955446809,134.122390675888,479.986437599388));
#61494=CARTESIAN_POINT('Ctrl Pts',(377.273115153633,133.687169688174,479.937413294597));
#61495=CARTESIAN_POINT('Ctrl Pts',(377.752122848375,133.359174868198,479.90264400738));
#61496=CARTESIAN_POINT('Ctrl Pts',(378.508507955966,132.602789760607,479.837256921998));
#61497=CARTESIAN_POINT('Ctrl Pts',(378.836500546947,132.123783304385,479.802374391123));
#61498=CARTESIAN_POINT('Ctrl Pts',(379.27171989715,131.073627786069,479.753090630837));
#61499=CARTESIAN_POINT('Ctrl Pts',(379.378917770959,130.502432883745,479.739413773764));
#61500=CARTESIAN_POINT('Ctrl Pts',(379.378917770959,129.966587529218,479.739413773764));
#61501=CARTESIAN_POINT('Origin',(375.11591777096,105.027992731211,473.546231028847));
#61502=CARTESIAN_POINT('',(379.37891777096,105.027992731211,467.092461505801));
#61503=CARTESIAN_POINT('Ctrl Pts',(379.37891777096,105.027992731211,467.092461505801));
#61504=CARTESIAN_POINT('Ctrl Pts',(379.37891777096,105.564673948596,467.092461505801));
#61505=CARTESIAN_POINT('Ctrl Pts',(379.271395654014,106.136215362734,467.114043744988));
#61506=CARTESIAN_POINT('Ctrl Pts',(378.835943832521,107.186131013358,467.191447285196));
#61507=CARTESIAN_POINT('Ctrl Pts',(378.50808272655,107.664620192018,467.246090869444));
#61508=CARTESIAN_POINT('Ctrl Pts',(377.752562213624,108.420140704944,467.348231142275));
#61509=CARTESIAN_POINT('Ctrl Pts',(377.274065797273,108.748015119979,467.402443514309));
#61510=CARTESIAN_POINT('Ctrl Pts',(376.224125087312,109.183476597627,467.478855729964));
#61511=CARTESIAN_POINT('Ctrl Pts',(375.652574862888,109.290992731211,467.500000551892));
#61512=CARTESIAN_POINT('Ctrl Pts',(374.579260679033,109.290992731211,467.500000551892));
#61513=CARTESIAN_POINT('Ctrl Pts',(374.007710454608,109.183476597627,467.478855729964));
#61514=CARTESIAN_POINT('Ctrl Pts',(372.957769744647,108.748015119978,467.402443514309));
#61515=CARTESIAN_POINT('Ctrl Pts',(372.479273328296,108.420140704943,467.348231142275));
#61516=CARTESIAN_POINT('Ctrl Pts',(371.723752815371,107.664620192018,467.246090869444));
#61517=CARTESIAN_POINT('Ctrl Pts',(371.395891709399,107.186131013357,467.191447285196));
#61518=CARTESIAN_POINT('Ctrl Pts',(370.960439887906,106.136215362734,467.114043744988));
#61519=CARTESIAN_POINT('Ctrl Pts',(370.852917770961,105.564673948595,467.092461505801));
#61520=CARTESIAN_POINT('Ctrl Pts',(370.852917770961,104.491311513826,467.092461505801));
#61521=CARTESIAN_POINT('Ctrl Pts',(370.960439887907,103.919770099687,467.114043744988));
#61522=CARTESIAN_POINT('Ctrl Pts',(371.3958917094,102.869854449064,467.191447285196));
#61523=CARTESIAN_POINT('Ctrl Pts',(371.723752815371,102.391365270404,467.246090869444));
#61524=CARTESIAN_POINT('Ctrl Pts',(372.479273328297,101.635844757478,467.348231142275));
#61525=CARTESIAN_POINT('Ctrl Pts',(372.957769744648,101.307970342443,467.402443514309));
#61526=CARTESIAN_POINT('Ctrl Pts',(374.007710454609,100.872508864795,467.478855729964));
#61527=CARTESIAN_POINT('Ctrl Pts',(374.579260679033,100.764992731211,467.500000551892));
#61528=CARTESIAN_POINT('Ctrl Pts',(375.652574862888,100.764992731211,467.500000551892));
#61529=CARTESIAN_POINT('Ctrl Pts',(376.224125087313,100.872508864795,467.478855729964));
#61530=CARTESIAN_POINT('Ctrl Pts',(377.274065797274,101.307970342443,467.402443514309));
#61531=CARTESIAN_POINT('Ctrl Pts',(377.752562213625,101.635844757479,467.348231142275));
#61532=CARTESIAN_POINT('Ctrl Pts',(378.50808272655,102.391365270404,467.246090869444));
#61533=CARTESIAN_POINT('Ctrl Pts',(378.835943832522,102.869854449064,467.191447285196));
#61534=CARTESIAN_POINT('Ctrl Pts',(379.271395654015,103.919770099688,467.114043744988));
#61535=CARTESIAN_POINT('Ctrl Pts',(379.378917770961,104.491311513827,467.092461505801));
#61536=CARTESIAN_POINT('Ctrl Pts',(379.37891777096,105.027992731211,467.092461505801));
#61537=CARTESIAN_POINT('',(379.37891777096,105.027992731211,479.739413773764));
#61538=CARTESIAN_POINT('',(379.37891777096,105.027992731211,473.546231028847));
#61539=CARTESIAN_POINT('Ctrl Pts',(379.37891777096,105.027992731211,479.739413773765));
#61540=CARTESIAN_POINT('Ctrl Pts',(379.37891777096,104.492147376685,479.739413773765));
#61541=CARTESIAN_POINT('Ctrl Pts',(379.271719897152,103.92095247436,479.753090630838));
#61542=CARTESIAN_POINT('Ctrl Pts',(378.836500546949,102.870796956045,479.802374391123));
#61543=CARTESIAN_POINT('Ctrl Pts',(378.508507955969,102.391790499823,479.837256921998));
#61544=CARTESIAN_POINT('Ctrl Pts',(377.752122848377,101.635405392231,479.90264400738));
#61545=CARTESIAN_POINT('Ctrl Pts',(377.273115153636,101.307410572254,479.937413294598));
#61546=CARTESIAN_POINT('Ctrl Pts',(376.222955446812,100.872189584541,479.986437599389));
#61547=CARTESIAN_POINT('Ctrl Pts',(375.651759093084,100.764992731211,480.000000551892));
#61548=CARTESIAN_POINT('Ctrl Pts',(374.580076448838,100.764992731211,480.000000551892));
#61549=CARTESIAN_POINT('Ctrl Pts',(374.00888009511,100.872189584541,479.986437599389));
#61550=CARTESIAN_POINT('Ctrl Pts',(372.958720388286,101.307410572254,479.937413294598));
#61551=CARTESIAN_POINT('Ctrl Pts',(372.479712693545,101.63540539223,479.90264400738));
#61552=CARTESIAN_POINT('Ctrl Pts',(371.723327585953,102.391790499822,479.837256921998));
#61553=CARTESIAN_POINT('Ctrl Pts',(371.395334994972,102.870796956044,479.802374391123));
#61554=CARTESIAN_POINT('Ctrl Pts',(370.960115644769,103.92095247436,479.753090630838));
#61555=CARTESIAN_POINT('Ctrl Pts',(370.852917770961,104.492147376684,479.739413773765));
#61556=CARTESIAN_POINT('Ctrl Pts',(370.852917770961,105.563838085737,479.739413773765));
#61557=CARTESIAN_POINT('Ctrl Pts',(370.960115644769,106.135032988061,479.753090630838));
#61558=CARTESIAN_POINT('Ctrl Pts',(371.395334994972,107.185188506377,479.802374391123));
#61559=CARTESIAN_POINT('Ctrl Pts',(371.723327585952,107.664194962599,479.837256921998));
#61560=CARTESIAN_POINT('Ctrl Pts',(372.479712693544,108.420580070191,479.90264400738));
#61561=CARTESIAN_POINT('Ctrl Pts',(372.958720388285,108.748574890167,479.937413294598));
#61562=CARTESIAN_POINT('Ctrl Pts',(374.008880095109,109.183795877881,479.986437599388));
#61563=CARTESIAN_POINT('Ctrl Pts',(374.580076448837,109.290992731211,480.000000551892));
#61564=CARTESIAN_POINT('Ctrl Pts',(375.651759093083,109.290992731211,480.000000551892));
#61565=CARTESIAN_POINT('Ctrl Pts',(376.222955446811,109.183795877881,479.986437599388));
#61566=CARTESIAN_POINT('Ctrl Pts',(377.273115153635,108.748574890168,479.937413294598));
#61567=CARTESIAN_POINT('Ctrl Pts',(377.752122848376,108.420580070191,479.90264400738));
#61568=CARTESIAN_POINT('Ctrl Pts',(378.508507955968,107.664194962599,479.837256921998));
#61569=CARTESIAN_POINT('Ctrl Pts',(378.836500546949,107.185188506377,479.802374391123));
#61570=CARTESIAN_POINT('Ctrl Pts',(379.271719897152,106.135032988062,479.753090630838));
#61571=CARTESIAN_POINT('Ctrl Pts',(379.37891777096,105.563838085738,479.739413773765));
#61572=CARTESIAN_POINT('Ctrl Pts',(379.37891777096,105.027992731211,479.739413773765));
#61573=CARTESIAN_POINT('Origin',(375.115917770963,70.0279927312109,462.203977458126));
#61574=CARTESIAN_POINT('',(378.505667770963,70.027992731211,469.769126393098));
#61575=CARTESIAN_POINT('',(378.505667770963,70.0279927312109,462.203977458126));
#61576=CARTESIAN_POINT('',(371.726167770963,70.0279927312108,469.769126393098));
#61577=CARTESIAN_POINT('Ctrl Pts',(371.726167770963,70.0279927312109,469.769126393098));
#61578=CARTESIAN_POINT('Ctrl Pts',(371.726167770963,70.4541839515356,469.769126393098));
#61579=CARTESIAN_POINT('Ctrl Pts',(371.811449811382,70.9084195073466,469.781261919919));
#61580=CARTESIAN_POINT('Ctrl Pts',(372.157548323688,71.7434257096236,469.82495721765));
#61581=CARTESIAN_POINT('Ctrl Pts',(372.418336416162,72.1242417994641,469.855870958313));
#61582=CARTESIAN_POINT('Ctrl Pts',(373.019665216239,72.7255705995408,469.913791149419));
#61583=CARTESIAN_POINT('Ctrl Pts',(373.400482816929,72.9863614255432,469.944580424309));
#61584=CARTESIAN_POINT('Ctrl Pts',(374.235494154767,73.3324619346181,469.987990393875));
#61585=CARTESIAN_POINT('Ctrl Pts',(374.689731492675,73.4177427312108,470.000000551892));
#61586=CARTESIAN_POINT('Ctrl Pts',(375.542104049251,73.4177427312109,470.000000551892));
#61587=CARTESIAN_POINT('Ctrl Pts',(375.996341387159,73.3324619346182,469.987990393875));
#61588=CARTESIAN_POINT('Ctrl Pts',(376.831352724996,72.9863614255434,469.944580424309));
#61589=CARTESIAN_POINT('Ctrl Pts',(377.212170325687,72.7255705995412,469.913791149419));
#61590=CARTESIAN_POINT('Ctrl Pts',(377.813499125764,72.1242417994645,469.855870958313));
#61591=CARTESIAN_POINT('Ctrl Pts',(378.074287218238,71.7434257096241,469.82495721765));
#61592=CARTESIAN_POINT('Ctrl Pts',(378.420385730544,70.9084195073471,469.781261919919));
#61593=CARTESIAN_POINT('Ctrl Pts',(378.505667770963,70.4541839515359,469.769126393098));
#61594=CARTESIAN_POINT('Ctrl Pts',(378.505667770963,70.0279927312111,469.769126393098));
#61595=CARTESIAN_POINT('Ctrl Pts',(378.505667770963,70.0279927312111,469.769126393098));
#61596=CARTESIAN_POINT('Ctrl Pts',(378.505667770963,69.6018015108863,469.769126393098));
#61597=CARTESIAN_POINT('Ctrl Pts',(378.420385730544,69.1475659550751,469.781261919919));
#61598=CARTESIAN_POINT('Ctrl Pts',(378.074287218238,68.3125597527981,469.82495721765));
#61599=CARTESIAN_POINT('Ctrl Pts',(377.813499125764,67.9317436629576,469.855870958313));
#61600=CARTESIAN_POINT('Ctrl Pts',(377.212170325687,67.3304148628808,469.913791149419));
#61601=CARTESIAN_POINT('Ctrl Pts',(376.831352724997,67.0696240368785,469.944580424309));
#61602=CARTESIAN_POINT('Ctrl Pts',(375.99634138716,66.7235235278036,469.987990393875));
#61603=CARTESIAN_POINT('Ctrl Pts',(375.542104049251,66.6382427312109,470.000000551892));
#61604=CARTESIAN_POINT('Ctrl Pts',(374.689731492675,66.6382427312108,470.000000551892));
#61605=CARTESIAN_POINT('Ctrl Pts',(374.235494154767,66.7235235278035,469.987990393875));
#61606=CARTESIAN_POINT('Ctrl Pts',(373.40048281693,67.0696240368783,469.944580424309));
#61607=CARTESIAN_POINT('Ctrl Pts',(373.019665216239,67.3304148628805,469.913791149419));
#61608=CARTESIAN_POINT('Ctrl Pts',(372.418336416162,67.9317436629572,469.855870958313));
#61609=CARTESIAN_POINT('Ctrl Pts',(372.157548323688,68.3125597527976,469.82495721765));
#61610=CARTESIAN_POINT('Ctrl Pts',(371.811449811382,69.1475659550746,469.781261919919));
#61611=CARTESIAN_POINT('Ctrl Pts',(371.726167770963,69.6018015108858,469.769126393098));
#61612=CARTESIAN_POINT('Ctrl Pts',(371.726167770963,70.0279927312106,469.769126393098));
#61613=CARTESIAN_POINT('Origin',(375.115917770964,55.0279927312109,462.203977458126));
#61614=CARTESIAN_POINT('',(378.505667770964,55.027992731211,469.769126393098));
#61615=CARTESIAN_POINT('',(378.505667770964,55.0279927312109,462.203977458126));
#61616=CARTESIAN_POINT('',(371.726167770964,55.0279927312099,469.769126393099));
#61617=CARTESIAN_POINT('Ctrl Pts',(371.726167770964,55.0279927312099,469.769126393098));
#61618=CARTESIAN_POINT('Ctrl Pts',(371.726167770964,55.4541839515347,469.769126393098));
#61619=CARTESIAN_POINT('Ctrl Pts',(371.811449811384,55.9084195073467,469.781261919919));
#61620=CARTESIAN_POINT('Ctrl Pts',(372.157548323689,56.7434257096237,469.82495721765));
#61621=CARTESIAN_POINT('Ctrl Pts',(372.418336416163,57.1242417994641,469.855870958314));
#61622=CARTESIAN_POINT('Ctrl Pts',(373.01966521624,57.7255705995409,469.913791149419));
#61623=CARTESIAN_POINT('Ctrl Pts',(373.40048281693,57.9863614255432,469.944580424309));
#61624=CARTESIAN_POINT('Ctrl Pts',(374.235494154768,58.3324619346181,469.987990393875));
#61625=CARTESIAN_POINT('Ctrl Pts',(374.689731492676,58.4177427312108,470.000000551892));
#61626=CARTESIAN_POINT('Ctrl Pts',(375.542104049252,58.4177427312109,470.000000551892));
#61627=CARTESIAN_POINT('Ctrl Pts',(375.99634138716,58.3324619346183,469.987990393875));
#61628=CARTESIAN_POINT('Ctrl Pts',(376.831352724997,57.9863614255434,469.944580424309));
#61629=CARTESIAN_POINT('Ctrl Pts',(377.212170325688,57.7255705995412,469.913791149419));
#61630=CARTESIAN_POINT('Ctrl Pts',(377.813499125765,57.1242417994645,469.855870958314));
#61631=CARTESIAN_POINT('Ctrl Pts',(378.074287218239,56.7434257096241,469.82495721765));
#61632=CARTESIAN_POINT('Ctrl Pts',(378.420385730545,55.9084195073471,469.781261919919));
#61633=CARTESIAN_POINT('Ctrl Pts',(378.505667770964,55.4541839515359,469.769126393098));
#61634=CARTESIAN_POINT('Ctrl Pts',(378.505667770964,55.0279927312111,469.769126393098));
#61635=CARTESIAN_POINT('Ctrl Pts',(378.505667770964,55.0279927312111,469.769126393098));
#61636=CARTESIAN_POINT('Ctrl Pts',(378.505667770964,54.6018015108864,469.769126393098));
#61637=CARTESIAN_POINT('Ctrl Pts',(378.420385730545,54.1475659550751,469.781261919919));
#61638=CARTESIAN_POINT('Ctrl Pts',(378.074287218239,53.3125597527981,469.82495721765));
#61639=CARTESIAN_POINT('Ctrl Pts',(377.813499125765,52.9317436629576,469.855870958314));
#61640=CARTESIAN_POINT('Ctrl Pts',(377.212170325688,52.3304148628809,469.913791149419));
#61641=CARTESIAN_POINT('Ctrl Pts',(376.831352724998,52.0696240368786,469.944580424309));
#61642=CARTESIAN_POINT('Ctrl Pts',(375.996341387161,51.7235235278036,469.987990393875));
#61643=CARTESIAN_POINT('Ctrl Pts',(375.542104049252,51.6382427312109,470.000000551892));
#61644=CARTESIAN_POINT('Ctrl Pts',(374.689731492677,51.6382427312109,470.000000551892));
#61645=CARTESIAN_POINT('Ctrl Pts',(374.235494154768,51.7235235278036,469.987990393875));
#61646=CARTESIAN_POINT('Ctrl Pts',(373.400482816931,52.0696240368784,469.944580424309));
#61647=CARTESIAN_POINT('Ctrl Pts',(373.01966521624,52.3304148628806,469.913791149419));
#61648=CARTESIAN_POINT('Ctrl Pts',(372.418336416164,52.9317436629573,469.855870958314));
#61649=CARTESIAN_POINT('Ctrl Pts',(372.157548323689,53.3125597527977,469.82495721765));
#61650=CARTESIAN_POINT('Ctrl Pts',(371.811449811384,54.1475659550746,469.781261919919));
#61651=CARTESIAN_POINT('Ctrl Pts',(371.726167770964,54.6018015108859,469.769126393098));
#61652=CARTESIAN_POINT('Ctrl Pts',(371.726167770964,55.0279927312106,469.769126393098));
#61653=CARTESIAN_POINT('Origin',(375.115917770961,95.0279927312111,422.490000551892));
#61654=CARTESIAN_POINT('',(397.615917770961,95.0279927312126,445.000000551892));
#61655=CARTESIAN_POINT('Origin',(375.115917770961,95.027992731211,445.000000551892));
#61656=CARTESIAN_POINT('Origin',(375.11591777096,120.027992731211,445.000000551892));
#61657=CARTESIAN_POINT('',(397.615917770958,145.027992731213,445.000000551892));
#61658=CARTESIAN_POINT('',(397.61591777096,120.027992731213,445.000000551892));
#61659=CARTESIAN_POINT('Origin',(375.115917770958,145.027992731211,445.000000551892));
#61660=CARTESIAN_POINT('Origin',(375.115917770963,67.527992731211,445.000000551892));
#61661=CARTESIAN_POINT('',(395.461568672241,50.0279927312126,459.527715079768));
#61662=CARTESIAN_POINT('',(400.115917770964,50.0279927312127,445.000000551893));
#61663=CARTESIAN_POINT('Origin',(375.115917770965,50.027992731211,445.000000551893));
#61664=CARTESIAN_POINT('Origin',(375.115917770965,50.027992731211,445.000000551893));
#61665=CARTESIAN_POINT('',(400.115917770962,85.027992731213,445.000000551892));
#61666=CARTESIAN_POINT('',(400.115917770963,67.5279927312129,445.000000551892));
#61667=CARTESIAN_POINT('',(354.770266869685,85.0279927312089,430.47228602402));
#61668=CARTESIAN_POINT('Origin',(375.115917770962,85.027992731211,445.000000551892));
#61669=CARTESIAN_POINT('Origin',(375.115917770962,85.027992731211,445.000000551892));
#61670=CARTESIAN_POINT('Origin',(375.115917770964,45.52799273121,445.000000551893));
#61671=CARTESIAN_POINT('',(391.392438491985,45.0279927312106,456.622172174192));
#61672=CARTESIAN_POINT('',(391.799351510011,45.527992731211,456.91272646475));
#61673=CARTESIAN_POINT('Origin',(375.115917770965,45.027992731211,445.000000551893));
#61674=CARTESIAN_POINT('Origin',(375.115917770965,45.0279927312111,424.990000551893));
#61675=CARTESIAN_POINT('Origin',(375.115917770958,144.527992731211,445.000000551892));
#61676=CARTESIAN_POINT('',(403.599829032745,140.027992731212,424.661200212869));
#61677=CARTESIAN_POINT('',(410.115917770958,140.027992731214,445.000000551892));
#61678=CARTESIAN_POINT('Origin',(375.115917770958,140.027992731211,445.000000551892));
#61679=CARTESIAN_POINT('Origin',(375.115917770958,140.027992731211,445.000000551892));
#61680=CARTESIAN_POINT('',(399.530698852489,145.027992731213,427.566743118444));
#61681=CARTESIAN_POINT('',(399.937611870515,144.527992731213,427.276188827887));
#61682=CARTESIAN_POINT('Origin',(375.115917770958,145.027992731211,445.000000551892));
#61683=CARTESIAN_POINT('Origin',(375.11591777096,117.52799273121,445.000000551892));
#61684=CARTESIAN_POINT('',(410.115917770961,95.027992731213,445.000000551892));
#61685=CARTESIAN_POINT('',(410.11591777096,117.527992731212,445.000000551892));
#61686=CARTESIAN_POINT('',(346.632006509173,95.0279927312094,424.66120021287));
#61687=CARTESIAN_POINT('Origin',(375.115917770961,95.027992731211,445.000000551892));
#61688=CARTESIAN_POINT('Origin',(375.115917770961,95.027992731211,445.000000551892));
#61689=CARTESIAN_POINT('Origin',(375.115917770958,145.027992731211,414.990000551892));
#61690=CARTESIAN_POINT('Origin',(375.115917770962,86.027992731211,445.000000551892));
#61691=CARTESIAN_POINT('',(353.956440833633,86.0279927312097,429.891177442905));
#61779=UNCERTAINTY_MEASURE_WITH_UNIT(LENGTH_MEASURE(0.01),#61812,
'DISTANCE_ACCURACY_VALUE',
'Maximum model space distance between geometric entities at asserted c
onnectivities');
#61780=UNCERTAINTY_MEASURE_WITH_UNIT(LENGTH_MEASURE(0.01),#61812,
'DISTANCE_ACCURACY_VALUE',
'Maximum model space distance between geometric entities at asserted c
onnectivities');
#61810=(
GEOMETRIC_REPRESENTATION_CONTEXT(3)
GLOBAL_UNCERTAINTY_ASSIGNED_CONTEXT((#61779))
GLOBAL_UNIT_ASSIGNED_CONTEXT((#61812,#61814,#61815))
REPRESENTATION_CONTEXT('','3D')
);
#61811=(
GEOMETRIC_REPRESENTATION_CONTEXT(3)
GLOBAL_UNCERTAINTY_ASSIGNED_CONTEXT((#61780))
GLOBAL_UNIT_ASSIGNED_CONTEXT((#61812,#61814,#61815))
REPRESENTATION_CONTEXT('','3D')
);
#61812=(
LENGTH_UNIT()
NAMED_UNIT(*)
SI_UNIT(.MILLI.,.METRE.)
);
#61814=(
NAMED_UNIT(*)
PLANE_ANGLE_UNIT()
SI_UNIT($,.RADIAN.)
);
#61815=(
NAMED_UNIT(*)
SI_UNIT($,.STERADIAN.)
SOLID_ANGLE_UNIT()
);
#61845=SHAPE_DEFINITION_REPRESENTATION(#61909,#61997);
#61909=PRODUCT_DEFINITION_SHAPE('',$,#62028);
#61997=SHAPE_REPRESENTATION('',(#38087),#61810);
#61998=PRODUCT_DEFINITION_CONTEXT('part definition',#62090,'design');
#62028=PRODUCT_DEFINITION('Shaft Coupling','Shaft Coupling',#62058,#61998);
#62058=PRODUCT_DEFINITION_FORMATION('',$,#62121);
#62090=APPLICATION_CONTEXT('Managed model based 3d engineering');
#62091=PRODUCT_CONTEXT('part definition',#62090,'mechanical');
#62121=PRODUCT('Shaft Coupling','Shaft Coupling',$,(#62091));
#62150=COLOUR_RGB('Grey',0.48,0.52,0.57);
#62151=FILL_AREA_STYLE_COLOUR('',#62150);
#62152=FILL_AREA_STYLE('',(#62151));
#62153=SURFACE_STYLE_FILL_AREA(#62152);
#62154=SURFACE_SIDE_STYLE('',(#62153));
#62155=SURFACE_STYLE_USAGE(.BOTH.,#62154);
#62156=PRESENTATION_STYLE_ASSIGNMENT((#62155));
ENDSEC;
END-ISO-10303-21;
